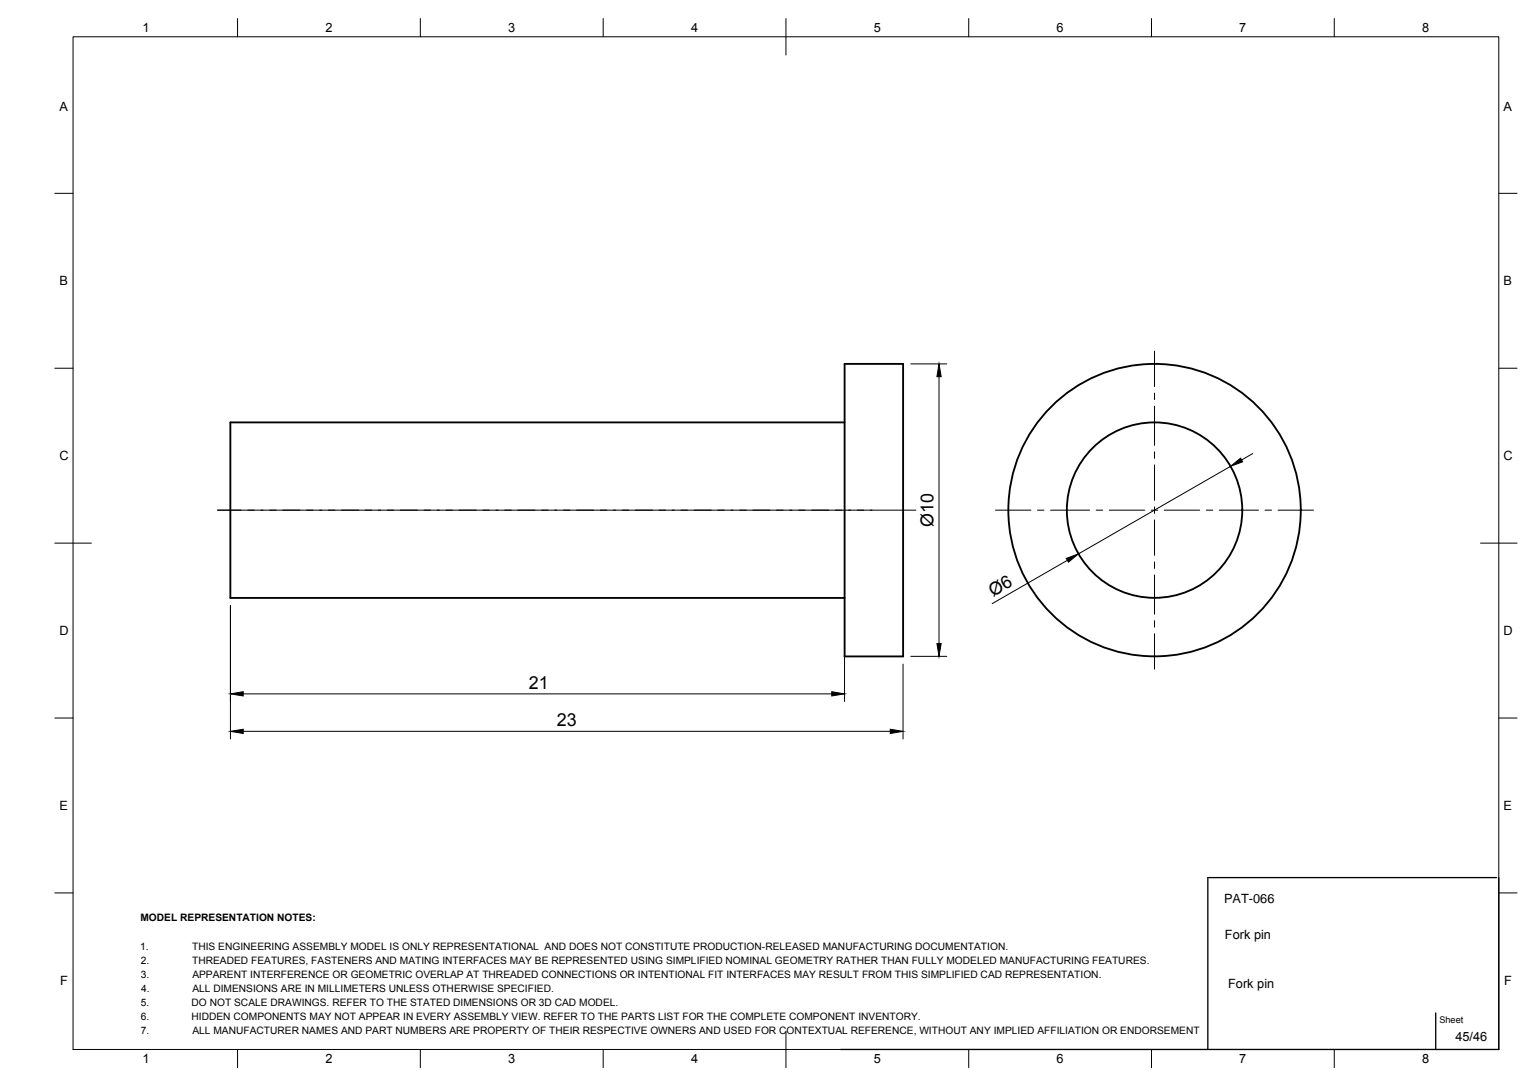
ISO-10303-21;
HEADER;
/* Generated by software containing ST-Developer
 * from STEP Tools, Inc. (www.steptools.com) 
 */

FILE_DESCRIPTION(
/* description */ ('Lever-operated bar clamp (toggle)'),
/* implementation_level */ '2;1');

FILE_NAME(
/* name */ 'Fork pin.step',
/* time_stamp */ '2026-10-28T03:25:02-07:00',
/* author */ (''),
/* organization */ (''),
/* preprocessor_version */ 'ST-DEVELOPER v20.2',
/* originating_system */ 'Autodesk Translation Framework v15.17.0.0',
/* authorisation */ '');

FILE_SCHEMA (('AUTOMOTIVE_DESIGN { 1 0 10303 214 3 1 1 }'));
ENDSEC;

DATA;
#10=MECHANICAL_DESIGN_GEOMETRIC_PRESENTATION_REPRESENTATION('',(#454),#12413);
#369=SHAPE_REPRESENTATION_RELATIONSHIP('SRR','None',#12613,#407);
#407=ADVANCED_BREP_SHAPE_REPRESENTATION('',(#497),#12410);
#454=STYLED_ITEM('',(#12869),#497);
#497=MANIFOLD_SOLID_BREP('Body1',#6617);
#649=FACE_BOUND('',#1830,.T.);
#874=PLANE('',#7854);
#875=PLANE('',#7859);
#876=PLANE('',#7862);
#1274=FACE_OUTER_BOUND('',#1829,.T.);
#1275=FACE_OUTER_BOUND('',#1831,.T.);
#1276=FACE_OUTER_BOUND('',#1832,.T.);
#1277=FACE_OUTER_BOUND('',#1833,.T.);
#1278=FACE_OUTER_BOUND('',#1834,.T.);
#1829=EDGE_LOOP('',(#5965));
#1830=EDGE_LOOP('',(#5966));
#1831=EDGE_LOOP('',(#5967,#5968,#5969,#5970));
#1832=EDGE_LOOP('',(#5971));
#1833=EDGE_LOOP('',(#5972,#5973,#5974,#5975));
#1834=EDGE_LOOP('',(#5976));
#2268=LINE('',#12243,#2709);
#2269=LINE('',#12249,#2710);
#2709=VECTOR('',#9949,0.5);
#2710=VECTOR('',#9958,0.3);
#3064=CIRCLE('',#7855,0.5);
#3065=CIRCLE('',#7856,0.3);
#3066=CIRCLE('',#7858,0.5);
#3067=CIRCLE('',#7861,0.3);
#3593=VERTEX_POINT('',#12237);
#3594=VERTEX_POINT('',#12239);
#3595=VERTEX_POINT('',#12242);
#3596=VERTEX_POINT('',#12247);
#4387=EDGE_CURVE('',#3593,#3593,#3064,.T.);
#4388=EDGE_CURVE('',#3594,#3594,#3065,.T.);
#4389=EDGE_CURVE('',#3593,#3595,#2268,.T.);
#4390=EDGE_CURVE('',#3595,#3595,#3066,.T.);
#4391=EDGE_CURVE('',#3596,#3596,#3067,.T.);
#4392=EDGE_CURVE('',#3596,#3594,#2269,.T.);
#5965=ORIENTED_EDGE('',*,*,#4387,.T.);
#5966=ORIENTED_EDGE('',*,*,#4388,.F.);
#5967=ORIENTED_EDGE('',*,*,#4387,.F.);
#5968=ORIENTED_EDGE('',*,*,#4389,.T.);
#5969=ORIENTED_EDGE('',*,*,#4390,.T.);
#5970=ORIENTED_EDGE('',*,*,#4389,.F.);
#5971=ORIENTED_EDGE('',*,*,#4390,.F.);
#5972=ORIENTED_EDGE('',*,*,#4391,.F.);
#5973=ORIENTED_EDGE('',*,*,#4392,.T.);
#5974=ORIENTED_EDGE('',*,*,#4388,.T.);
#5975=ORIENTED_EDGE('',*,*,#4392,.F.);
#5976=ORIENTED_EDGE('',*,*,#4391,.T.);
#6159=CYLINDRICAL_SURFACE('',#7857,0.5);
#6160=CYLINDRICAL_SURFACE('',#7860,0.3);
#6549=ADVANCED_FACE('',(#1274,#649),#874,.T.);
#6550=ADVANCED_FACE('',(#1275),#6159,.T.);
#6551=ADVANCED_FACE('',(#1276),#875,.F.);
#6552=ADVANCED_FACE('',(#1277),#6160,.T.);
#6553=ADVANCED_FACE('',(#1278),#876,.T.);
#6617=CLOSED_SHELL('',(#6549,#6550,#6551,#6552,#6553));
#7853=AXIS2_PLACEMENT_3D('',#12235,#9939,#9940);
#7854=AXIS2_PLACEMENT_3D('',#12236,#9941,#9942);
#7855=AXIS2_PLACEMENT_3D('',#12238,#9943,#9944);
#7856=AXIS2_PLACEMENT_3D('',#12240,#9945,#9946);
#7857=AXIS2_PLACEMENT_3D('',#12241,#9947,#9948);
#7858=AXIS2_PLACEMENT_3D('',#12244,#9950,#9951);
#7859=AXIS2_PLACEMENT_3D('',#12245,#9952,#9953);
#7860=AXIS2_PLACEMENT_3D('',#12246,#9954,#9955);
#7861=AXIS2_PLACEMENT_3D('',#12248,#9956,#9957);
#7862=AXIS2_PLACEMENT_3D('',#12250,#9959,#9960);
#9939=DIRECTION('axis',(0.,0.,1.));
#9940=DIRECTION('refdir',(1.,0.,0.));
#9941=DIRECTION('center_axis',(0.,1.,0.));
#9942=DIRECTION('ref_axis',(1.,0.,0.));
#9943=DIRECTION('center_axis',(0.,1.,0.));
#9944=DIRECTION('ref_axis',(1.,0.,0.));
#9945=DIRECTION('center_axis',(0.,1.,0.));
#9946=DIRECTION('ref_axis',(1.,0.,0.));
#9947=DIRECTION('center_axis',(0.,1.,0.));
#9948=DIRECTION('ref_axis',(1.,0.,0.));
#9949=DIRECTION('',(0.,-1.,0.));
#9950=DIRECTION('center_axis',(0.,1.,0.));
#9951=DIRECTION('ref_axis',(1.,0.,0.));
#9952=DIRECTION('center_axis',(0.,1.,0.));
#9953=DIRECTION('ref_axis',(1.,0.,0.));
#9954=DIRECTION('center_axis',(0.,1.,0.));
#9955=DIRECTION('ref_axis',(1.,0.,0.));
#9956=DIRECTION('center_axis',(0.,1.,0.));
#9957=DIRECTION('ref_axis',(1.,0.,0.));
#9958=DIRECTION('',(0.,-1.,0.));
#9959=DIRECTION('center_axis',(0.,1.,0.));
#9960=DIRECTION('ref_axis',(1.,0.,0.));
#12235=CARTESIAN_POINT('',(0.,0.,0.));
#12236=CARTESIAN_POINT('Origin',(0.,-6.,4.668081457105));
#12237=CARTESIAN_POINT('',(-0.5,-6.,4.668081457105));
#12238=CARTESIAN_POINT('Origin',(0.,-6.,4.668081457105));
#12239=CARTESIAN_POINT('',(-0.3,-6.,4.668081457105));
#12240=CARTESIAN_POINT('Origin',(0.,-6.,4.668081457105));
#12241=CARTESIAN_POINT('Origin',(0.,-6.2,4.668081457105));
#12242=CARTESIAN_POINT('',(-0.5,-6.2,4.668081457105));
#12243=CARTESIAN_POINT('',(-0.5,-6.2,4.668081457105));
#12244=CARTESIAN_POINT('Origin',(0.,-6.2,4.668081457105));
#12245=CARTESIAN_POINT('Origin',(0.,-6.2,4.668081457105));
#12246=CARTESIAN_POINT('Origin',(0.,-6.,4.668081457105));
#12247=CARTESIAN_POINT('',(-0.3,-3.9,4.668081457105));
#12248=CARTESIAN_POINT('Origin',(0.,-3.9,4.668081457105));
#12249=CARTESIAN_POINT('',(-0.3,-6.,4.668081457105));
#12250=CARTESIAN_POINT('Origin',(0.,-3.9,4.668081457105));
#12364=UNCERTAINTY_MEASURE_WITH_UNIT(LENGTH_MEASURE(0.001),#12414,
'DISTANCE_ACCURACY_VALUE',
'Maximum model space distance between geometric entities at asserted c
onnectivities');
#12367=UNCERTAINTY_MEASURE_WITH_UNIT(LENGTH_MEASURE(0.001),#12414,
'DISTANCE_ACCURACY_VALUE',
'Maximum model space distance between geometric entities at asserted c
onnectivities');
#12410=(
GEOMETRIC_REPRESENTATION_CONTEXT(3)
GLOBAL_UNCERTAINTY_ASSIGNED_CONTEXT((#12364))
GLOBAL_UNIT_ASSIGNED_CONTEXT((#12414,#12416,#12417))
REPRESENTATION_CONTEXT('','3D')
);
#12413=(
GEOMETRIC_REPRESENTATION_CONTEXT(3)
GLOBAL_UNCERTAINTY_ASSIGNED_CONTEXT((#12367))
GLOBAL_UNIT_ASSIGNED_CONTEXT((#12414,#12416,#12417))
REPRESENTATION_CONTEXT('','3D')
);
#12414=(
LENGTH_UNIT()
NAMED_UNIT(*)
SI_UNIT(.CENTI.,.METRE.)
);
#12416=(
NAMED_UNIT(*)
PLANE_ANGLE_UNIT()
SI_UNIT($,.RADIAN.)
);
#12417=(
NAMED_UNIT(*)
SI_UNIT($,.STERADIAN.)
SOLID_ANGLE_UNIT()
);
#12460=SHAPE_DEFINITION_REPRESENTATION(#12560,#12613);
#12560=PRODUCT_DEFINITION_SHAPE('',$,#12659);
#12613=SHAPE_REPRESENTATION('',(#7853),#12410);
#12616=PRODUCT_DEFINITION_CONTEXT('part definition',#12753,'design');
#12659=PRODUCT_DEFINITION('Fork pin','Fork pin',#12704,#12616);
#12704=PRODUCT_DEFINITION_FORMATION('',$,#12797);
#12753=APPLICATION_CONTEXT(
'Core Data for Automotive Mechanical Design Process');
#12754=PRODUCT_CONTEXT('part definition',#12753,'mechanical');
#12797=PRODUCT('Fork pin','Fork pin','Fork pin',(#12754));
#12863=COLOUR_RGB('Grey',0.48,0.52,0.57);
#12864=FILL_AREA_STYLE_COLOUR('',#12863);
#12865=FILL_AREA_STYLE('',(#12864));
#12866=SURFACE_STYLE_FILL_AREA(#12865);
#12867=SURFACE_SIDE_STYLE('',(#12866));
#12868=SURFACE_STYLE_USAGE(.BOTH.,#12867);
#12869=PRESENTATION_STYLE_ASSIGNMENT((#12868));
ENDSEC;
END-ISO-10303-21;
